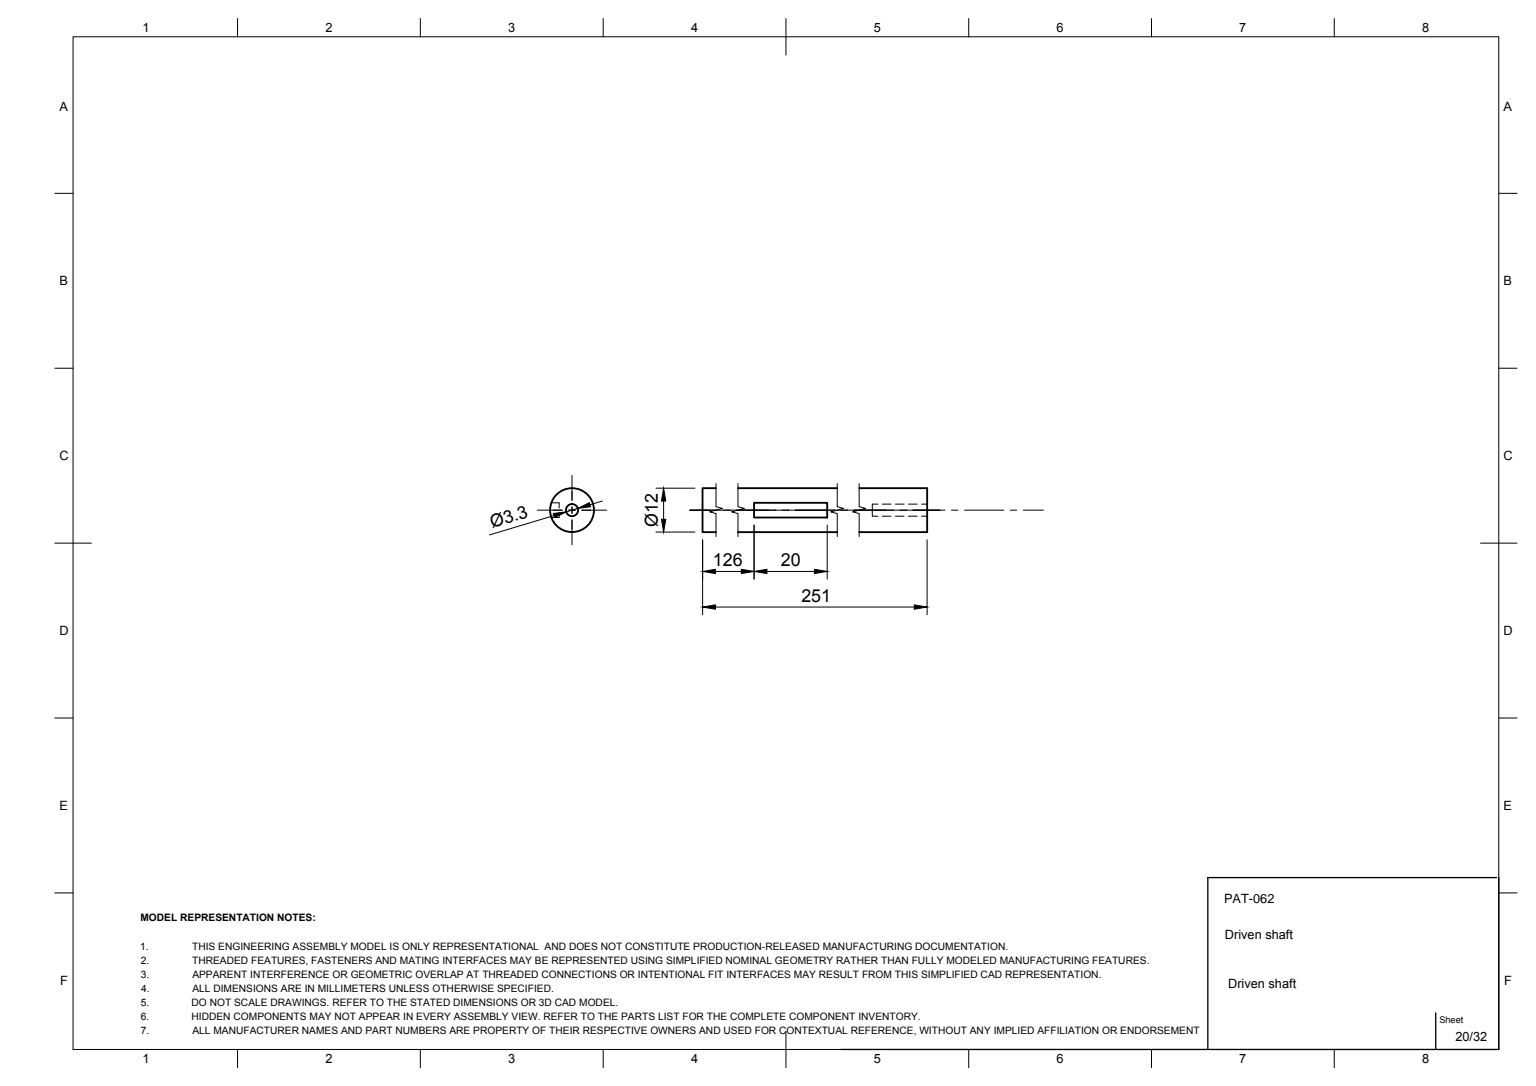
ISO-10303-21;
HEADER;
/* Generated by software containing ST-Developer
 * from STEP Tools, Inc. (www.steptools.com) 
 */

FILE_DESCRIPTION(
/* description */ ('Jaw-coupled motor to shaft test stand'),
/* implementation_level */ '2;1');

FILE_NAME(
/* name */ 'Driven shaft.step',
/* time_stamp */ '2026-10-27T10:46:06-07:00',
/* author */ (''),
/* organization */ (''),
/* preprocessor_version */ 'ST-DEVELOPER v20.2',
/* originating_system */ 'Autodesk Translation Framework v15.17.0.0',
/* authorisation */ '');

FILE_SCHEMA (('AUTOMOTIVE_DESIGN { 1 0 10303 214 3 1 1 }'));
ENDSEC;

DATA;
#10=MECHANICAL_DESIGN_GEOMETRIC_PRESENTATION_REPRESENTATION('',(#359),#19361);
#294=SHAPE_REPRESENTATION_RELATIONSHIP('SRR','None',#19510,#326);
#326=ADVANCED_BREP_SHAPE_REPRESENTATION('',(#390),#19346);
#359=STYLED_ITEM('',(#19746),#390);
#390=MANIFOLD_SOLID_BREP('Body1',#11005);
#483=FACE_BOUND('',#1931,.T.);
#484=FACE_BOUND('',#1933,.T.);
#652=PLANE('',#11744);
#653=PLANE('',#11745);
#654=PLANE('',#11747);
#655=PLANE('',#11748);
#656=PLANE('',#11749);
#657=PLANE('',#11754);
#658=PLANE('',#11758);
#659=PLANE('',#11759);
#1223=FACE_OUTER_BOUND('',#1923,.T.);
#1224=FACE_OUTER_BOUND('',#1924,.T.);
#1225=FACE_OUTER_BOUND('',#1925,.T.);
#1226=FACE_OUTER_BOUND('',#1926,.T.);
#1227=FACE_OUTER_BOUND('',#1927,.T.);
#1228=FACE_OUTER_BOUND('',#1928,.T.);
#1229=FACE_OUTER_BOUND('',#1929,.T.);
#1230=FACE_OUTER_BOUND('',#1930,.T.);
#1231=FACE_OUTER_BOUND('',#1932,.T.);
#1232=FACE_OUTER_BOUND('',#1934,.T.);
#1923=EDGE_LOOP('',(#8212,#8213,#8214,#8215));
#1924=EDGE_LOOP('',(#8216,#8217,#8218,#8219));
#1925=EDGE_LOOP('',(#8220,#8221,#8222,#8223));
#1926=EDGE_LOOP('',(#8224,#8225,#8226,#8227));
#1927=EDGE_LOOP('',(#8228,#8229,#8230,#8231));
#1928=EDGE_LOOP('',(#8232,#8233,#8234,#8235));
#1929=EDGE_LOOP('',(#8236));
#1930=EDGE_LOOP('',(#8237,#8238,#8239,#8240));
#1931=EDGE_LOOP('',(#8241,#8242,#8243,#8244));
#1932=EDGE_LOOP('',(#8245));
#1933=EDGE_LOOP('',(#8246));
#1934=EDGE_LOOP('',(#8247));
#2664=LINE('',#16816,#3817);
#2665=LINE('',#16818,#3818);
#2666=LINE('',#16820,#3819);
#2667=LINE('',#16821,#3820);
#2668=LINE('',#16826,#3821);
#2669=LINE('',#16827,#3822);
#2670=LINE('',#16830,#3823);
#2671=LINE('',#16832,#3824);
#2672=LINE('',#16833,#3825);
#2673=LINE('',#16835,#3826);
#2674=LINE('',#16842,#3827);
#2675=LINE('',#16849,#3828);
#3817=VECTOR('',#13373,1.);
#3818=VECTOR('',#13374,1.);
#3819=VECTOR('',#13375,1.);
#3820=VECTOR('',#13376,1.);
#3821=VECTOR('',#13381,1.);
#3822=VECTOR('',#13382,1.);
#3823=VECTOR('',#13385,1.);
#3824=VECTOR('',#13386,1.);
#3825=VECTOR('',#13387,1.);
#3826=VECTOR('',#13390,1.);
#3827=VECTOR('',#13399,0.165);
#3828=VECTOR('',#13408,0.6);
#4801=CIRCLE('',#11746,0.6);
#4802=CIRCLE('',#11750,0.6);
#4803=CIRCLE('',#11752,0.165);
#4804=CIRCLE('',#11753,0.165);
#4805=CIRCLE('',#11756,0.6);
#4806=CIRCLE('',#11757,0.6);
#5237=VERTEX_POINT('',#16814);
#5238=VERTEX_POINT('',#16815);
#5239=VERTEX_POINT('',#16817);
#5240=VERTEX_POINT('',#16819);
#5241=VERTEX_POINT('',#16823);
#5242=VERTEX_POINT('',#16825);
#5243=VERTEX_POINT('',#16829);
#5244=VERTEX_POINT('',#16831);
#5245=VERTEX_POINT('',#16839);
#5246=VERTEX_POINT('',#16841);
#5247=VERTEX_POINT('',#16846);
#5248=VERTEX_POINT('',#16848);
#6317=EDGE_CURVE('',#5237,#5238,#2664,.T.);
#6318=EDGE_CURVE('',#5237,#5239,#2665,.T.);
#6319=EDGE_CURVE('',#5240,#5239,#2666,.T.);
#6320=EDGE_CURVE('',#5240,#5238,#2667,.T.);
#6321=EDGE_CURVE('',#5238,#5241,#4801,.T.);
#6322=EDGE_CURVE('',#5242,#5240,#2668,.T.);
#6323=EDGE_CURVE('',#5241,#5242,#2669,.T.);
#6324=EDGE_CURVE('',#5241,#5243,#2670,.T.);
#6325=EDGE_CURVE('',#5242,#5244,#2671,.T.);
#6326=EDGE_CURVE('',#5244,#5243,#2672,.T.);
#6327=EDGE_CURVE('',#5239,#5244,#2673,.T.);
#6328=EDGE_CURVE('',#5243,#5237,#4802,.T.);
#6329=EDGE_CURVE('',#5245,#5245,#4803,.T.);
#6330=EDGE_CURVE('',#5245,#5246,#2674,.T.);
#6331=EDGE_CURVE('',#5246,#5246,#4804,.T.);
#6332=EDGE_CURVE('',#5247,#5247,#4805,.T.);
#6333=EDGE_CURVE('',#5247,#5248,#2675,.T.);
#6334=EDGE_CURVE('',#5248,#5248,#4806,.T.);
#8212=ORIENTED_EDGE('',*,*,#6317,.F.);
#8213=ORIENTED_EDGE('',*,*,#6318,.T.);
#8214=ORIENTED_EDGE('',*,*,#6319,.F.);
#8215=ORIENTED_EDGE('',*,*,#6320,.T.);
#8216=ORIENTED_EDGE('',*,*,#6321,.F.);
#8217=ORIENTED_EDGE('',*,*,#6320,.F.);
#8218=ORIENTED_EDGE('',*,*,#6322,.F.);
#8219=ORIENTED_EDGE('',*,*,#6323,.F.);
#8220=ORIENTED_EDGE('',*,*,#6324,.F.);
#8221=ORIENTED_EDGE('',*,*,#6323,.T.);
#8222=ORIENTED_EDGE('',*,*,#6325,.T.);
#8223=ORIENTED_EDGE('',*,*,#6326,.T.);
#8224=ORIENTED_EDGE('',*,*,#6322,.T.);
#8225=ORIENTED_EDGE('',*,*,#6319,.T.);
#8226=ORIENTED_EDGE('',*,*,#6327,.T.);
#8227=ORIENTED_EDGE('',*,*,#6325,.F.);
#8228=ORIENTED_EDGE('',*,*,#6328,.F.);
#8229=ORIENTED_EDGE('',*,*,#6326,.F.);
#8230=ORIENTED_EDGE('',*,*,#6327,.F.);
#8231=ORIENTED_EDGE('',*,*,#6318,.F.);
#8232=ORIENTED_EDGE('',*,*,#6329,.F.);
#8233=ORIENTED_EDGE('',*,*,#6330,.T.);
#8234=ORIENTED_EDGE('',*,*,#6331,.F.);
#8235=ORIENTED_EDGE('',*,*,#6330,.F.);
#8236=ORIENTED_EDGE('',*,*,#6329,.T.);
#8237=ORIENTED_EDGE('',*,*,#6332,.F.);
#8238=ORIENTED_EDGE('',*,*,#6333,.T.);
#8239=ORIENTED_EDGE('',*,*,#6334,.T.);
#8240=ORIENTED_EDGE('',*,*,#6333,.F.);
#8241=ORIENTED_EDGE('',*,*,#6324,.T.);
#8242=ORIENTED_EDGE('',*,*,#6328,.T.);
#8243=ORIENTED_EDGE('',*,*,#6317,.T.);
#8244=ORIENTED_EDGE('',*,*,#6321,.T.);
#8245=ORIENTED_EDGE('',*,*,#6332,.T.);
#8246=ORIENTED_EDGE('',*,*,#6331,.T.);
#8247=ORIENTED_EDGE('',*,*,#6334,.F.);
#10327=CYLINDRICAL_SURFACE('',#11751,0.165);
#10328=CYLINDRICAL_SURFACE('',#11755,0.6);
#10565=ADVANCED_FACE('',(#1223),#652,.F.);
#10566=ADVANCED_FACE('',(#1224),#653,.T.);
#10567=ADVANCED_FACE('',(#1225),#654,.F.);
#10568=ADVANCED_FACE('',(#1226),#655,.F.);
#10569=ADVANCED_FACE('',(#1227),#656,.F.);
#10570=ADVANCED_FACE('',(#1228),#10327,.F.);
#10571=ADVANCED_FACE('',(#1229),#657,.T.);
#10572=ADVANCED_FACE('',(#1230,#483),#10328,.T.);
#10573=ADVANCED_FACE('',(#1231,#484),#658,.T.);
#10574=ADVANCED_FACE('',(#1232),#659,.F.);
#11005=CLOSED_SHELL('',(#10565,#10566,#10567,#10568,#10569,#10570,#10571,
#10572,#10573,#10574));
#11743=AXIS2_PLACEMENT_3D('',#16812,#13369,#13370);
#11744=AXIS2_PLACEMENT_3D('',#16813,#13371,#13372);
#11745=AXIS2_PLACEMENT_3D('',#16822,#13377,#13378);
#11746=AXIS2_PLACEMENT_3D('',#16824,#13379,#13380);
#11747=AXIS2_PLACEMENT_3D('',#16828,#13383,#13384);
#11748=AXIS2_PLACEMENT_3D('',#16834,#13388,#13389);
#11749=AXIS2_PLACEMENT_3D('',#16836,#13391,#13392);
#11750=AXIS2_PLACEMENT_3D('',#16837,#13393,#13394);
#11751=AXIS2_PLACEMENT_3D('',#16838,#13395,#13396);
#11752=AXIS2_PLACEMENT_3D('',#16840,#13397,#13398);
#11753=AXIS2_PLACEMENT_3D('',#16843,#13400,#13401);
#11754=AXIS2_PLACEMENT_3D('',#16844,#13402,#13403);
#11755=AXIS2_PLACEMENT_3D('',#16845,#13404,#13405);
#11756=AXIS2_PLACEMENT_3D('',#16847,#13406,#13407);
#11757=AXIS2_PLACEMENT_3D('',#16850,#13409,#13410);
#11758=AXIS2_PLACEMENT_3D('',#16851,#13411,#13412);
#11759=AXIS2_PLACEMENT_3D('',#16852,#13413,#13414);
#13369=DIRECTION('axis',(0.,0.,1.));
#13370=DIRECTION('refdir',(1.,0.,0.));
#13371=DIRECTION('center_axis',(-1.,0.,0.));
#13372=DIRECTION('ref_axis',(0.,0.,1.));
#13373=DIRECTION('',(0.,-1.,0.));
#13374=DIRECTION('',(0.,0.,1.));
#13375=DIRECTION('',(0.,1.,0.));
#13376=DIRECTION('',(0.,0.,-1.));
#13377=DIRECTION('center_axis',(0.,1.,0.));
#13378=DIRECTION('ref_axis',(1.,0.,0.));
#13379=DIRECTION('center_axis',(0.,-1.,0.));
#13380=DIRECTION('ref_axis',(1.,0.,0.));
#13381=DIRECTION('',(-1.,0.,0.));
#13382=DIRECTION('',(0.,0.,1.));
#13383=DIRECTION('center_axis',(1.,0.,0.));
#13384=DIRECTION('ref_axis',(0.,0.,-1.));
#13385=DIRECTION('',(0.,1.,0.));
#13386=DIRECTION('',(0.,1.,0.));
#13387=DIRECTION('',(0.,0.,-1.));
#13388=DIRECTION('center_axis',(0.,0.,1.));
#13389=DIRECTION('ref_axis',(1.,0.,0.));
#13390=DIRECTION('',(1.,0.,0.));
#13391=DIRECTION('center_axis',(0.,1.,0.));
#13392=DIRECTION('ref_axis',(0.,0.,1.));
#13393=DIRECTION('center_axis',(0.,1.,0.));
#13394=DIRECTION('ref_axis',(1.,0.,0.));
#13395=DIRECTION('center_axis',(0.,1.,0.));
#13396=DIRECTION('ref_axis',(1.,0.,0.));
#13397=DIRECTION('center_axis',(0.,1.,0.));
#13398=DIRECTION('ref_axis',(1.,0.,0.));
#13399=DIRECTION('',(0.,1.,0.));
#13400=DIRECTION('center_axis',(0.,-1.,0.));
#13401=DIRECTION('ref_axis',(1.,0.,0.));
#13402=DIRECTION('center_axis',(0.,1.,0.));
#13403=DIRECTION('ref_axis',(1.,0.,0.));
#13404=DIRECTION('center_axis',(0.,1.,0.));
#13405=DIRECTION('ref_axis',(1.,0.,0.));
#13406=DIRECTION('center_axis',(0.,1.,0.));
#13407=DIRECTION('ref_axis',(1.,0.,0.));
#13408=DIRECTION('',(0.,-1.,0.));
#13409=DIRECTION('center_axis',(0.,1.,0.));
#13410=DIRECTION('ref_axis',(1.,0.,0.));
#13411=DIRECTION('center_axis',(0.,1.,0.));
#13412=DIRECTION('ref_axis',(1.,0.,0.));
#13413=DIRECTION('center_axis',(0.,1.,0.));
#13414=DIRECTION('ref_axis',(1.,0.,0.));
#16812=CARTESIAN_POINT('',(0.,0.,0.));
#16813=CARTESIAN_POINT('Origin',(-0.2,9.5,3.52));
#16814=CARTESIAN_POINT('',(-0.2,11.5,3.65431457505076));
#16815=CARTESIAN_POINT('',(-0.2,9.5,3.65431457505076));
#16816=CARTESIAN_POINT('',(-0.2,-3.1,3.65431457505076));
#16817=CARTESIAN_POINT('',(-0.2,11.5,3.87));
#16818=CARTESIAN_POINT('',(-0.2,11.5,3.87));
#16819=CARTESIAN_POINT('',(-0.2,9.5,3.87));
#16820=CARTESIAN_POINT('',(-0.2,9.5,3.87));
#16821=CARTESIAN_POINT('',(-0.2,9.5,3.87));
#16822=CARTESIAN_POINT('Origin',(0.,9.5,3.695));
#16823=CARTESIAN_POINT('',(0.2,9.5,3.65431457505076));
#16824=CARTESIAN_POINT('Origin',(0.,9.5,4.22));
#16825=CARTESIAN_POINT('',(0.2,9.5,3.87));
#16826=CARTESIAN_POINT('',(0.2,9.5,3.87));
#16827=CARTESIAN_POINT('',(0.2,9.5,3.52));
#16828=CARTESIAN_POINT('Origin',(0.2,9.5,3.87));
#16829=CARTESIAN_POINT('',(0.2,11.5,3.65431457505076));
#16830=CARTESIAN_POINT('',(0.2,-3.1,3.65431457505076));
#16831=CARTESIAN_POINT('',(0.2,11.5,3.87));
#16832=CARTESIAN_POINT('',(0.2,9.5,3.87));
#16833=CARTESIAN_POINT('',(0.2,11.5,3.52));
#16834=CARTESIAN_POINT('Origin',(-0.2,9.5,3.87));
#16835=CARTESIAN_POINT('',(0.2,11.5,3.87));
#16836=CARTESIAN_POINT('Origin',(0.,11.5,3.695));
#16837=CARTESIAN_POINT('Origin',(0.,11.5,4.22));
#16838=CARTESIAN_POINT('Origin',(0.,20.5,4.22));
#16839=CARTESIAN_POINT('',(-0.165,20.5,4.22));
#16840=CARTESIAN_POINT('Origin',(0.,20.5,4.22));
#16841=CARTESIAN_POINT('',(-0.165,22.,4.22));
#16842=CARTESIAN_POINT('',(-0.165,20.5,4.22));
#16843=CARTESIAN_POINT('Origin',(0.,22.,4.22));
#16844=CARTESIAN_POINT('Origin',(0.,20.5,4.22));
#16845=CARTESIAN_POINT('Origin',(0.,-3.1,4.22));
#16846=CARTESIAN_POINT('',(-0.6,22.,4.22));
#16847=CARTESIAN_POINT('Origin',(0.,22.,4.22));
#16848=CARTESIAN_POINT('',(-0.6,-3.1,4.22));
#16849=CARTESIAN_POINT('',(-0.6,-3.1,4.22));
#16850=CARTESIAN_POINT('Origin',(0.,-3.1,4.22));
#16851=CARTESIAN_POINT('Origin',(0.,22.,4.22));
#16852=CARTESIAN_POINT('Origin',(0.,-3.1,4.22));
#19308=UNCERTAINTY_MEASURE_WITH_UNIT(LENGTH_MEASURE(0.001),#19362,
'DISTANCE_ACCURACY_VALUE',
'Maximum model space distance between geometric entities at asserted c
onnectivities');
#19323=UNCERTAINTY_MEASURE_WITH_UNIT(LENGTH_MEASURE(0.001),#19362,
'DISTANCE_ACCURACY_VALUE',
'Maximum model space distance between geometric entities at asserted c
onnectivities');
#19346=(
GEOMETRIC_REPRESENTATION_CONTEXT(3)
GLOBAL_UNCERTAINTY_ASSIGNED_CONTEXT((#19308))
GLOBAL_UNIT_ASSIGNED_CONTEXT((#19362,#19364,#19365))
REPRESENTATION_CONTEXT('','3D')
);
#19361=(
GEOMETRIC_REPRESENTATION_CONTEXT(3)
GLOBAL_UNCERTAINTY_ASSIGNED_CONTEXT((#19323))
GLOBAL_UNIT_ASSIGNED_CONTEXT((#19362,#19364,#19365))
REPRESENTATION_CONTEXT('','3D')
);
#19362=(
LENGTH_UNIT()
NAMED_UNIT(*)
SI_UNIT(.CENTI.,.METRE.)
);
#19364=(
NAMED_UNIT(*)
PLANE_ANGLE_UNIT()
SI_UNIT($,.RADIAN.)
);
#19365=(
NAMED_UNIT(*)
SI_UNIT($,.STERADIAN.)
SOLID_ANGLE_UNIT()
);
#19388=SHAPE_DEFINITION_REPRESENTATION(#19452,#19510);
#19452=PRODUCT_DEFINITION_SHAPE('',$,#19548);
#19510=SHAPE_REPRESENTATION('',(#11743),#19346);
#19525=PRODUCT_DEFINITION_CONTEXT('part definition',#19638,'design');
#19548=PRODUCT_DEFINITION('Driven shaft','Driven shaft',#19585,#19525);
#19585=PRODUCT_DEFINITION_FORMATION('',$,#19662);
#19638=APPLICATION_CONTEXT(
'Core Data for Automotive Mechanical Design Process');
#19639=PRODUCT_CONTEXT('part definition',#19638,'mechanical');
#19662=PRODUCT('Driven shaft','Driven shaft','Driven shaft',(#19639));
#19740=COLOUR_RGB('Grey',0.48,0.52,0.57);
#19741=FILL_AREA_STYLE_COLOUR('',#19740);
#19742=FILL_AREA_STYLE('',(#19741));
#19743=SURFACE_STYLE_FILL_AREA(#19742);
#19744=SURFACE_SIDE_STYLE('',(#19743));
#19745=SURFACE_STYLE_USAGE(.BOTH.,#19744);
#19746=PRESENTATION_STYLE_ASSIGNMENT((#19745));
ENDSEC;
END-ISO-10303-21;
